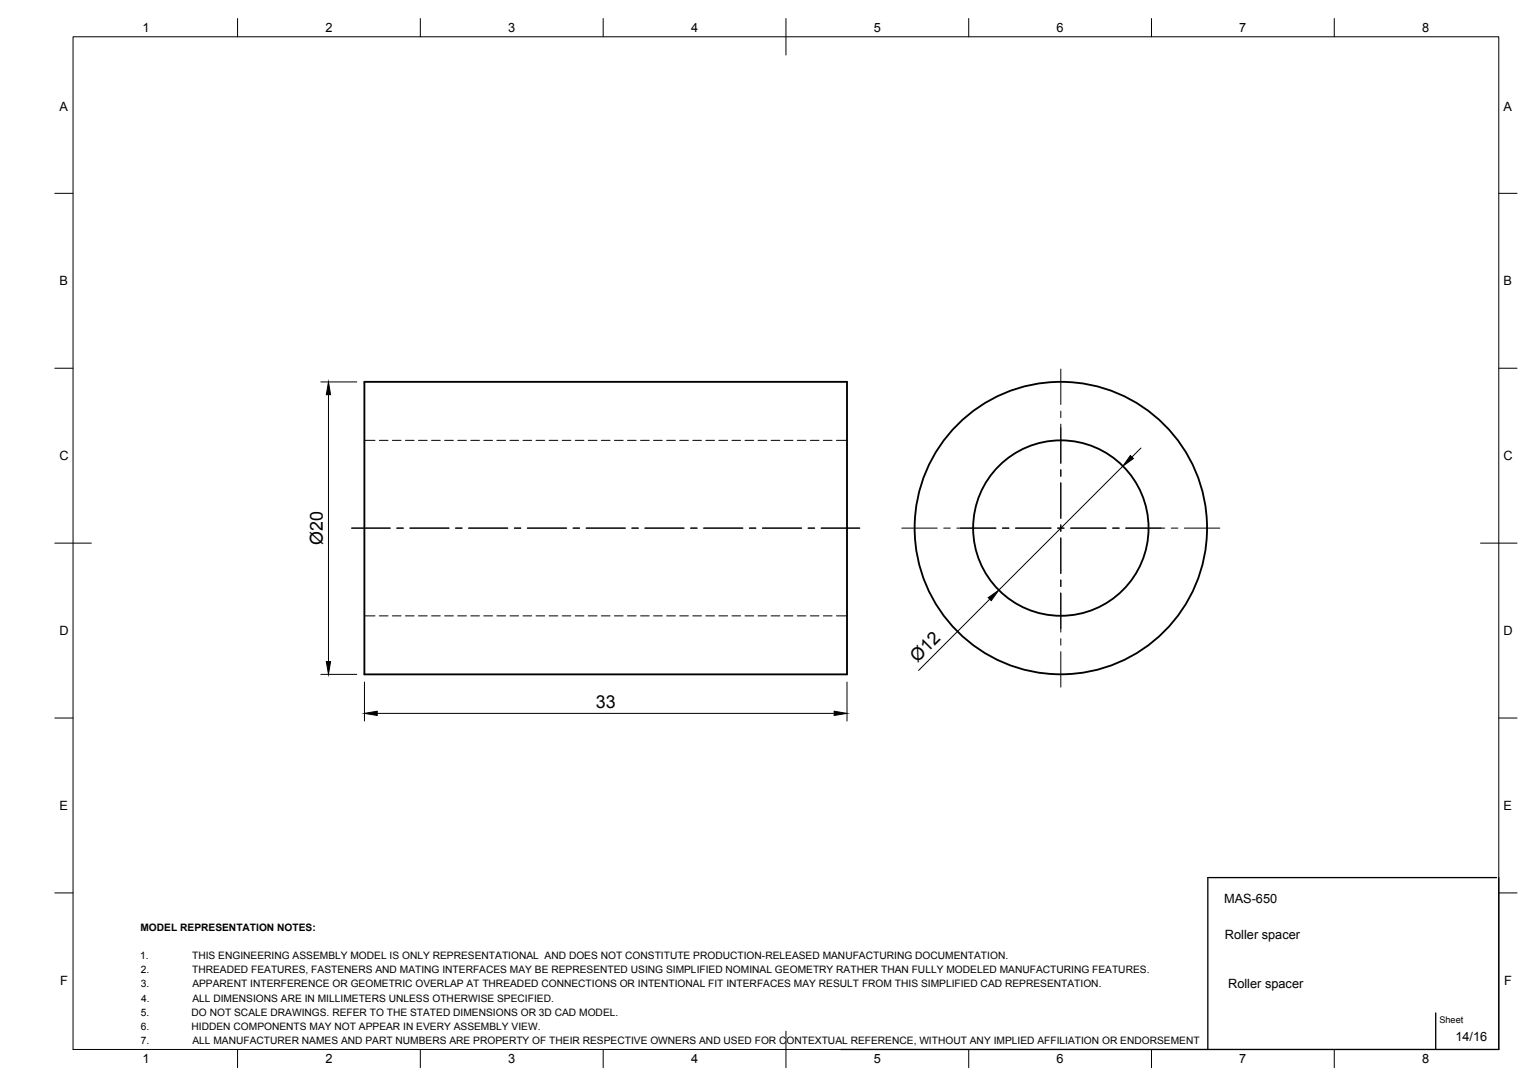
ISO-10303-21;
HEADER;
/* Generated by software containing ST-Developer
 * from STEP Tools, Inc. (www.steptools.com) 
 */

FILE_DESCRIPTION(
/* description */ ('Independent manual traversing gantry with native reusable aluminum pr
ofiles,180mm captured carriage travel, four bronze-bushed rollers, lin
ked ideal rolling motion, bonded acetal lateral guides, positive welde
d end stops and fully retained axle stacks. Editable native profile cu
t lengths220/400mm. Tool attachments viaM6 bridge-plate taps; mounted 
tool outside assembly. Welds, anchors, adhesives, fits, traction, load
/speed/structural/life ratings unassigned.'),
/* implementation_level */ '2;1');

FILE_NAME(
/* name */ 'Roller spacer.step',
/* time_stamp */ '2026-11-09T20:04:38-08:00',
/* author */ (''),
/* organization */ (''),
/* preprocessor_version */ 'ST-DEVELOPER v20.2',
/* originating_system */ 'Autodesk Translation Framework v15.17.0.0',
/* authorisation */ '');

FILE_SCHEMA (('AUTOMOTIVE_DESIGN { 1 0 10303 214 3 1 1 }'));
ENDSEC;

DATA;
#10=MECHANICAL_DESIGN_GEOMETRIC_PRESENTATION_REPRESENTATION('',(#484),#13231);
#452=SHAPE_REPRESENTATION_RELATIONSHIP('SRR','None',#13341,#468);
#468=ADVANCED_BREP_SHAPE_REPRESENTATION('',(#500),#13228);
#484=STYLED_ITEM('',(#13422),#500);
#500=MANIFOLD_SOLID_BREP('Body1',#4164);
#546=FACE_BOUND('',#1109,.T.);
#547=FACE_BOUND('',#1111,.T.);
#627=PLANE('',#4658);
#628=PLANE('',#4659);
#842=FACE_OUTER_BOUND('',#1106,.T.);
#843=FACE_OUTER_BOUND('',#1107,.T.);
#844=FACE_OUTER_BOUND('',#1108,.T.);
#845=FACE_OUTER_BOUND('',#1110,.T.);
#1106=EDGE_LOOP('',(#3762,#3763,#3764,#3765));
#1107=EDGE_LOOP('',(#3766,#3767,#3768,#3769));
#1108=EDGE_LOOP('',(#3770));
#1109=EDGE_LOOP('',(#3771));
#1110=EDGE_LOOP('',(#3772));
#1111=EDGE_LOOP('',(#3773));
#1380=LINE('',#13099,#1642);
#1381=LINE('',#13105,#1643);
#1642=VECTOR('',#5611,6.);
#1643=VECTOR('',#5618,10.);
#1740=CIRCLE('',#4653,6.);
#1741=CIRCLE('',#4654,6.);
#1742=CIRCLE('',#4656,10.);
#1743=CIRCLE('',#4657,10.);
#2112=VERTEX_POINT('',#13096);
#2113=VERTEX_POINT('',#13098);
#2114=VERTEX_POINT('',#13102);
#2115=VERTEX_POINT('',#13104);
#2664=EDGE_CURVE('',#2112,#2112,#1740,.T.);
#2665=EDGE_CURVE('',#2112,#2113,#1380,.T.);
#2666=EDGE_CURVE('',#2113,#2113,#1741,.T.);
#2667=EDGE_CURVE('',#2114,#2114,#1742,.T.);
#2668=EDGE_CURVE('',#2114,#2115,#1381,.T.);
#2669=EDGE_CURVE('',#2115,#2115,#1743,.T.);
#3762=ORIENTED_EDGE('',*,*,#2664,.F.);
#3763=ORIENTED_EDGE('',*,*,#2665,.T.);
#3764=ORIENTED_EDGE('',*,*,#2666,.T.);
#3765=ORIENTED_EDGE('',*,*,#2665,.F.);
#3766=ORIENTED_EDGE('',*,*,#2667,.F.);
#3767=ORIENTED_EDGE('',*,*,#2668,.T.);
#3768=ORIENTED_EDGE('',*,*,#2669,.T.);
#3769=ORIENTED_EDGE('',*,*,#2668,.F.);
#3770=ORIENTED_EDGE('',*,*,#2667,.T.);
#3771=ORIENTED_EDGE('',*,*,#2664,.T.);
#3772=ORIENTED_EDGE('',*,*,#2669,.F.);
#3773=ORIENTED_EDGE('',*,*,#2666,.F.);
#3924=CYLINDRICAL_SURFACE('',#4652,6.);
#3925=CYLINDRICAL_SURFACE('',#4655,10.);
#4139=ADVANCED_FACE('',(#842),#3924,.F.);
#4140=ADVANCED_FACE('',(#843),#3925,.T.);
#4141=ADVANCED_FACE('',(#844,#546),#627,.T.);
#4142=ADVANCED_FACE('',(#845,#547),#628,.F.);
#4164=CLOSED_SHELL('',(#4139,#4140,#4141,#4142));
#4651=AXIS2_PLACEMENT_3D('',#13094,#5605,#5606);
#4652=AXIS2_PLACEMENT_3D('',#13095,#5607,#5608);
#4653=AXIS2_PLACEMENT_3D('',#13097,#5609,#5610);
#4654=AXIS2_PLACEMENT_3D('',#13100,#5612,#5613);
#4655=AXIS2_PLACEMENT_3D('',#13101,#5614,#5615);
#4656=AXIS2_PLACEMENT_3D('',#13103,#5616,#5617);
#4657=AXIS2_PLACEMENT_3D('',#13106,#5619,#5620);
#4658=AXIS2_PLACEMENT_3D('',#13107,#5621,#5622);
#4659=AXIS2_PLACEMENT_3D('',#13108,#5623,#5624);
#5605=DIRECTION('axis',(0.,0.,1.));
#5606=DIRECTION('refdir',(1.,0.,0.));
#5607=DIRECTION('center_axis',(0.,0.,1.));
#5608=DIRECTION('ref_axis',(1.,0.,0.));
#5609=DIRECTION('center_axis',(0.,0.,-1.));
#5610=DIRECTION('ref_axis',(1.,0.,0.));
#5611=DIRECTION('',(0.,0.,-1.));
#5612=DIRECTION('center_axis',(0.,0.,-1.));
#5613=DIRECTION('ref_axis',(1.,0.,0.));
#5614=DIRECTION('center_axis',(0.,0.,1.));
#5615=DIRECTION('ref_axis',(1.,0.,0.));
#5616=DIRECTION('center_axis',(0.,0.,1.));
#5617=DIRECTION('ref_axis',(1.,0.,0.));
#5618=DIRECTION('',(0.,0.,-1.));
#5619=DIRECTION('center_axis',(0.,0.,1.));
#5620=DIRECTION('ref_axis',(1.,0.,0.));
#5621=DIRECTION('center_axis',(0.,0.,1.));
#5622=DIRECTION('ref_axis',(1.,0.,0.));
#5623=DIRECTION('center_axis',(0.,0.,1.));
#5624=DIRECTION('ref_axis',(1.,0.,0.));
#13094=CARTESIAN_POINT('',(0.,0.,0.));
#13095=CARTESIAN_POINT('Origin',(0.,0.,0.));
#13096=CARTESIAN_POINT('',(-6.,-7.34788079488412E-16,33.));
#13097=CARTESIAN_POINT('Origin',(0.,0.,33.));
#13098=CARTESIAN_POINT('',(-6.,-7.34788079488412E-16,0.));
#13099=CARTESIAN_POINT('',(-6.,-7.34788079488412E-16,0.));
#13100=CARTESIAN_POINT('Origin',(0.,0.,0.));
#13101=CARTESIAN_POINT('Origin',(0.,0.,0.));
#13102=CARTESIAN_POINT('',(-10.,-1.22464679914735E-15,33.));
#13103=CARTESIAN_POINT('Origin',(0.,0.,33.));
#13104=CARTESIAN_POINT('',(-10.,-1.22464679914735E-15,0.));
#13105=CARTESIAN_POINT('',(-10.,-1.22464679914735E-15,0.));
#13106=CARTESIAN_POINT('Origin',(0.,0.,0.));
#13107=CARTESIAN_POINT('Origin',(0.,0.,33.));
#13108=CARTESIAN_POINT('Origin',(0.,0.,0.));
#13210=UNCERTAINTY_MEASURE_WITH_UNIT(LENGTH_MEASURE(0.01),#13232,
'DISTANCE_ACCURACY_VALUE',
'Maximum model space distance between geometric entities at asserted c
onnectivities');
#13213=UNCERTAINTY_MEASURE_WITH_UNIT(LENGTH_MEASURE(0.01),#13232,
'DISTANCE_ACCURACY_VALUE',
'Maximum model space distance between geometric entities at asserted c
onnectivities');
#13228=(
GEOMETRIC_REPRESENTATION_CONTEXT(3)
GLOBAL_UNCERTAINTY_ASSIGNED_CONTEXT((#13210))
GLOBAL_UNIT_ASSIGNED_CONTEXT((#13232,#13234,#13235))
REPRESENTATION_CONTEXT('','3D')
);
#13231=(
GEOMETRIC_REPRESENTATION_CONTEXT(3)
GLOBAL_UNCERTAINTY_ASSIGNED_CONTEXT((#13213))
GLOBAL_UNIT_ASSIGNED_CONTEXT((#13232,#13234,#13235))
REPRESENTATION_CONTEXT('','3D')
);
#13232=(
LENGTH_UNIT()
NAMED_UNIT(*)
SI_UNIT(.MILLI.,.METRE.)
);
#13234=(
NAMED_UNIT(*)
PLANE_ANGLE_UNIT()
SI_UNIT($,.RADIAN.)
);
#13235=(
NAMED_UNIT(*)
SI_UNIT($,.STERADIAN.)
SOLID_ANGLE_UNIT()
);
#13250=SHAPE_DEFINITION_REPRESENTATION(#13267,#13341);
#13267=PRODUCT_DEFINITION_SHAPE('',$,#13359);
#13341=SHAPE_REPRESENTATION('',(#4651),#13228);
#13344=PRODUCT_DEFINITION_CONTEXT('part definition',#13397,'design');
#13359=PRODUCT_DEFINITION('Roller spacer','Roller spacer',#13376,#13344);
#13376=PRODUCT_DEFINITION_FORMATION('',$,#13413);
#13397=APPLICATION_CONTEXT(
'Core Data for Automotive Mechanical Design Process');
#13398=PRODUCT_CONTEXT('part definition',#13397,'mechanical');
#13413=PRODUCT('Roller spacer','Roller spacer',$,(#13398));
#13422=PRESENTATION_STYLE_ASSIGNMENT((#13436));
#13436=SURFACE_STYLE_USAGE(.BOTH.,#13450);
#13450=SURFACE_SIDE_STYLE('',(#13464));
#13464=SURFACE_STYLE_FILL_AREA(#13478);
#13478=FILL_AREA_STYLE('Gray',(#13492));
#13492=FILL_AREA_STYLE_COLOUR('Gray',#13506);
#13506=COLOUR_RGB('Gray',0.407843137254902,0.447058823529412,0.498039215686275);
ENDSEC;
END-ISO-10303-21;
